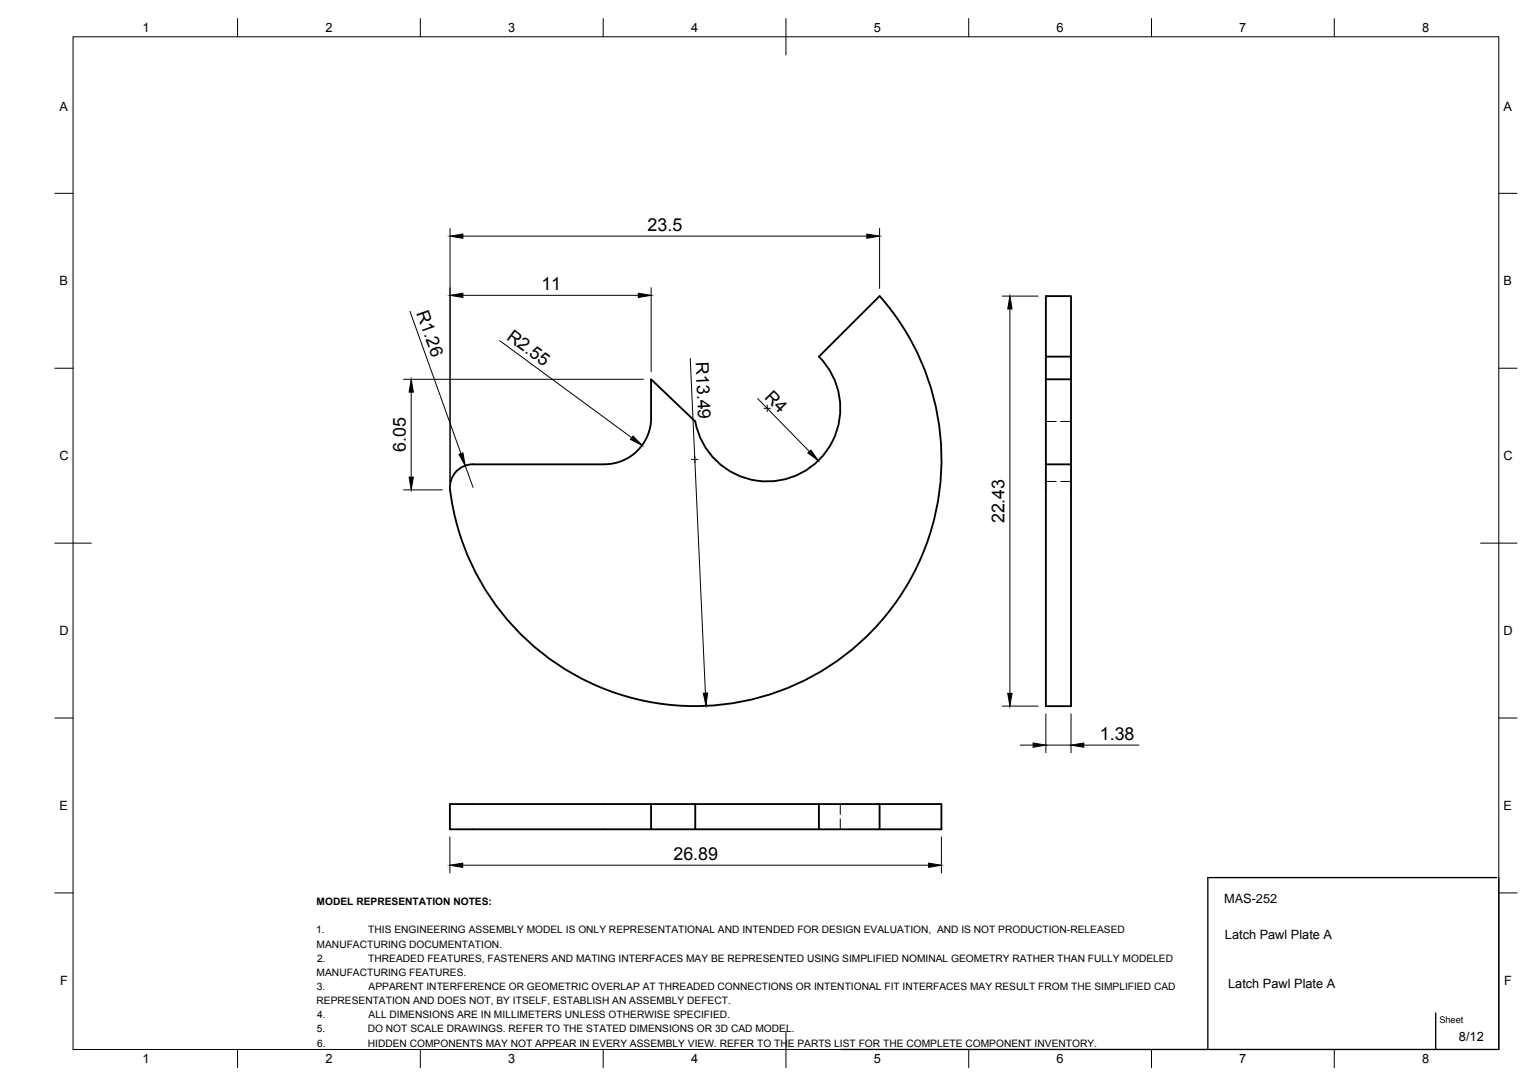
ISO-10303-21;
HEADER;
FILE_DESCRIPTION((''),'2;1');
FILE_NAME('Latch Pawl Plate A.step','2026-10-06T07:01:46+05:00',(''),(''),'','','');
FILE_SCHEMA (('AUTOMOTIVE_DESIGN { 1 0 10303 214 3 1 1 }'));
ENDSEC;
DATA;
#10=MECHANICAL_DESIGN_GEOMETRIC_PRESENTATION_REPRESENTATION('',(#150),#11396);
#120=SHAPE_REPRESENTATION_RELATIONSHIP('SRR','None',#11467,#135) ;
#135=ADVANCED_BREP_SHAPE_REPRESENTATION('',(#165),#11393) ;
#150=STYLED_ITEM('',(#11551),#165) ;
#165=MANIFOLD_SOLID_BREP('Latch Pawl Plate A',#5581) ;
#494=PLANE('',#6342) ;
#495=PLANE('',#6343) ;
#496=PLANE('',#6347) ;
#497=PLANE('',#6354) ;
#498=PLANE('',#6355) ;
#499=PLANE('',#6356) ;
#817=FACE_OUTER_BOUND('',#1190,.T.) ;
#818=FACE_OUTER_BOUND('',#1191,.T.) ;
#819=FACE_OUTER_BOUND('',#1192,.T.) ;
#820=FACE_OUTER_BOUND('',#1193,.T.) ;
#821=FACE_OUTER_BOUND('',#1194,.T.) ;
#822=FACE_OUTER_BOUND('',#1195,.T.) ;
#823=FACE_OUTER_BOUND('',#1196,.T.) ;
#824=FACE_OUTER_BOUND('',#1197,.T.) ;
#825=FACE_OUTER_BOUND('',#1198,.T.) ;
#826=FACE_OUTER_BOUND('',#1199,.T.) ;
#1190=EDGE_LOOP('',(#4966,#4967,#4968,#4969)) ;
#1191=EDGE_LOOP('',(#4970,#4971,#4972,#4973)) ;
#1192=EDGE_LOOP('',(#4974,#4975,#4976,#4977)) ;
#1193=EDGE_LOOP('',(#4978,#4979,#4980,#4981)) ;
#1194=EDGE_LOOP('',(#4982,#4983,#4984,#4985)) ;
#1195=EDGE_LOOP('',(#4986,#4987,#4988,#4989)) ;
#1196=EDGE_LOOP('',(#4990,#4991,#4992,#4993)) ;
#1197=EDGE_LOOP('',(#4994,#4995,#4996,#4997)) ;
#1198=EDGE_LOOP('',(#4998,#4999,#5000,#5001,#5002,#5003,#5004,#5005)) ;
#1199=EDGE_LOOP('',(#5006,#5007,#5008,#5009,#5010,#5011,#5012,#5013)) ;
#1567=LINE('',#11213,#1950) ;
#1568=LINE('',#11216,#1951) ;
#1569=LINE('',#11219,#1952) ;
#1570=LINE('',#11221,#1953) ;
#1571=LINE('',#11222,#1954) ;
#1572=LINE('',#11225,#1955) ;
#1573=LINE('',#11227,#1956) ;
#1574=LINE('',#11228,#1957) ;
#1575=LINE('',#11234,#1958) ;
#1576=LINE('',#11237,#1959) ;
#1577=LINE('',#11239,#1960) ;
#1578=LINE('',#11240,#1961) ;
#1579=LINE('',#11246,#1962) ;
#1580=LINE('',#11252,#1963) ;
#1581=LINE('',#11254,#1964) ;
#1582=LINE('',#11255,#1965) ;
#1950=VECTOR('',#7943,10.) ;
#1951=VECTOR('',#7946,10.) ;
#1952=VECTOR('',#7949,10.) ;
#1953=VECTOR('',#7950,10.) ;
#1954=VECTOR('',#7951,10.) ;
#1955=VECTOR('',#7954,10.) ;
#1956=VECTOR('',#7955,10.) ;
#1957=VECTOR('',#7956,10.) ;
#1958=VECTOR('',#7963,10.) ;
#1959=VECTOR('',#7966,10.) ;
#1960=VECTOR('',#7967,10.) ;
#1961=VECTOR('',#7968,10.) ;
#1962=VECTOR('',#7975,10.) ;
#1963=VECTOR('',#7982,10.) ;
#1964=VECTOR('',#7985,10.) ;
#1965=VECTOR('',#7986,10.) ;
#2243=CIRCLE('',#6340,2.55000000000001) ;
#2244=CIRCLE('',#6341,2.55000000000001) ;
#2245=CIRCLE('',#6345,4.00044834860818) ;
#2246=CIRCLE('',#6346,4.00044834860818) ;
#2247=CIRCLE('',#6349,13.4930018479188) ;
#2248=CIRCLE('',#6350,13.4930018479188) ;
#2249=CIRCLE('',#6352,1.26348906976575) ;
#2250=CIRCLE('',#6353,1.26348906976575) ;
#2704=VERTEX_POINT('',#11209) ;
#2705=VERTEX_POINT('',#11210) ;
#2706=VERTEX_POINT('',#11212) ;
#2707=VERTEX_POINT('',#11214) ;
#2708=VERTEX_POINT('',#11218) ;
#2709=VERTEX_POINT('',#11220) ;
#2710=VERTEX_POINT('',#11224) ;
#2711=VERTEX_POINT('',#11226) ;
#2712=VERTEX_POINT('',#11230) ;
#2713=VERTEX_POINT('',#11232) ;
#2714=VERTEX_POINT('',#11236) ;
#2715=VERTEX_POINT('',#11238) ;
#2716=VERTEX_POINT('',#11242) ;
#2717=VERTEX_POINT('',#11244) ;
#2718=VERTEX_POINT('',#11248) ;
#2719=VERTEX_POINT('',#11250) ;
#3465=EDGE_CURVE('',#2704,#2705,#2243,.T.) ;
#3466=EDGE_CURVE('',#2704,#2706,#1567,.T.) ;
#3467=EDGE_CURVE('',#2707,#2706,#2244,.T.) ;
#3468=EDGE_CURVE('',#2705,#2707,#1568,.T.) ;
#3469=EDGE_CURVE('',#2708,#2705,#1569,.T.) ;
#3470=EDGE_CURVE('',#2709,#2707,#1570,.T.) ;
#3471=EDGE_CURVE('',#2708,#2709,#1571,.T.) ;
#3472=EDGE_CURVE('',#2710,#2708,#1572,.T.) ;
#3473=EDGE_CURVE('',#2711,#2709,#1573,.T.) ;
#3474=EDGE_CURVE('',#2710,#2711,#1574,.T.) ;
#3475=EDGE_CURVE('',#2710,#2712,#2245,.T.) ;
#3476=EDGE_CURVE('',#2713,#2711,#2246,.T.) ;
#3477=EDGE_CURVE('',#2712,#2713,#1575,.T.) ;
#3478=EDGE_CURVE('',#2714,#2712,#1576,.T.) ;
#3479=EDGE_CURVE('',#2715,#2713,#1577,.T.) ;
#3480=EDGE_CURVE('',#2714,#2715,#1578,.T.) ;
#3481=EDGE_CURVE('',#2716,#2714,#2247,.T.) ;
#3482=EDGE_CURVE('',#2717,#2715,#2248,.T.) ;
#3483=EDGE_CURVE('',#2716,#2717,#1579,.T.) ;
#3484=EDGE_CURVE('',#2718,#2716,#2249,.T.) ;
#3485=EDGE_CURVE('',#2719,#2717,#2250,.T.) ;
#3486=EDGE_CURVE('',#2718,#2719,#1580,.T.) ;
#3487=EDGE_CURVE('',#2704,#2718,#1581,.T.) ;
#3488=EDGE_CURVE('',#2706,#2719,#1582,.T.) ;
#4966=ORIENTED_EDGE('',*,*,#3465,.F.) ;
#4967=ORIENTED_EDGE('',*,*,#3466,.T.) ;
#4968=ORIENTED_EDGE('',*,*,#3467,.F.) ;
#4969=ORIENTED_EDGE('',*,*,#3468,.F.) ;
#4970=ORIENTED_EDGE('',*,*,#3469,.T.) ;
#4971=ORIENTED_EDGE('',*,*,#3468,.T.) ;
#4972=ORIENTED_EDGE('',*,*,#3470,.F.) ;
#4973=ORIENTED_EDGE('',*,*,#3471,.F.) ;
#4974=ORIENTED_EDGE('',*,*,#3472,.T.) ;
#4975=ORIENTED_EDGE('',*,*,#3471,.T.) ;
#4976=ORIENTED_EDGE('',*,*,#3473,.F.) ;
#4977=ORIENTED_EDGE('',*,*,#3474,.F.) ;
#4978=ORIENTED_EDGE('',*,*,#3475,.F.) ;
#4979=ORIENTED_EDGE('',*,*,#3474,.T.) ;
#4980=ORIENTED_EDGE('',*,*,#3476,.F.) ;
#4981=ORIENTED_EDGE('',*,*,#3477,.F.) ;
#4982=ORIENTED_EDGE('',*,*,#3478,.T.) ;
#4983=ORIENTED_EDGE('',*,*,#3477,.T.) ;
#4984=ORIENTED_EDGE('',*,*,#3479,.F.) ;
#4985=ORIENTED_EDGE('',*,*,#3480,.F.) ;
#4986=ORIENTED_EDGE('',*,*,#3481,.T.) ;
#4987=ORIENTED_EDGE('',*,*,#3480,.T.) ;
#4988=ORIENTED_EDGE('',*,*,#3482,.F.) ;
#4989=ORIENTED_EDGE('',*,*,#3483,.F.) ;
#4990=ORIENTED_EDGE('',*,*,#3484,.T.) ;
#4991=ORIENTED_EDGE('',*,*,#3483,.T.) ;
#4992=ORIENTED_EDGE('',*,*,#3485,.F.) ;
#4993=ORIENTED_EDGE('',*,*,#3486,.F.) ;
#4994=ORIENTED_EDGE('',*,*,#3487,.T.) ;
#4995=ORIENTED_EDGE('',*,*,#3486,.T.) ;
#4996=ORIENTED_EDGE('',*,*,#3488,.F.) ;
#4997=ORIENTED_EDGE('',*,*,#3466,.F.) ;
#4998=ORIENTED_EDGE('',*,*,#3488,.T.) ;
#4999=ORIENTED_EDGE('',*,*,#3485,.T.) ;
#5000=ORIENTED_EDGE('',*,*,#3482,.T.) ;
#5001=ORIENTED_EDGE('',*,*,#3479,.T.) ;
#5002=ORIENTED_EDGE('',*,*,#3476,.T.) ;
#5003=ORIENTED_EDGE('',*,*,#3473,.T.) ;
#5004=ORIENTED_EDGE('',*,*,#3470,.T.) ;
#5005=ORIENTED_EDGE('',*,*,#3467,.T.) ;
#5006=ORIENTED_EDGE('',*,*,#3487,.F.) ;
#5007=ORIENTED_EDGE('',*,*,#3465,.T.) ;
#5008=ORIENTED_EDGE('',*,*,#3469,.F.) ;
#5009=ORIENTED_EDGE('',*,*,#3472,.F.) ;
#5010=ORIENTED_EDGE('',*,*,#3475,.T.) ;
#5011=ORIENTED_EDGE('',*,*,#3478,.F.) ;
#5012=ORIENTED_EDGE('',*,*,#3481,.F.) ;
#5013=ORIENTED_EDGE('',*,*,#3484,.F.) ;
#5220=CYLINDRICAL_SURFACE('',#6339,2.55000000000001) ;
#5221=CYLINDRICAL_SURFACE('',#6344,4.00044834860818) ;
#5222=CYLINDRICAL_SURFACE('',#6348,13.4930018479188) ;
#5223=CYLINDRICAL_SURFACE('',#6351,1.26348906976575) ;
#5542=ADVANCED_FACE('',(#817),#5220,.F.) ;
#5543=ADVANCED_FACE('',(#818),#494,.T.) ;
#5544=ADVANCED_FACE('',(#819),#495,.T.) ;
#5545=ADVANCED_FACE('',(#820),#5221,.F.) ;
#5546=ADVANCED_FACE('',(#821),#496,.T.) ;
#5547=ADVANCED_FACE('',(#822),#5222,.T.) ;
#5548=ADVANCED_FACE('',(#823),#5223,.T.) ;
#5549=ADVANCED_FACE('',(#824),#497,.T.) ;
#5550=ADVANCED_FACE('',(#825),#498,.T.) ;
#5551=ADVANCED_FACE('',(#826),#499,.F.) ;
#5581=CLOSED_SHELL('',(#5542,#5543,#5544,#5545,#5546,#5547,#5548,#5549,
#5550,#5551)) ;
#6338=AXIS2_PLACEMENT_3D('',#11207,#7937,#7938) ;
#6339=AXIS2_PLACEMENT_3D('',#11208,#7939,#7940) ;
#6340=AXIS2_PLACEMENT_3D('',#11211,#7941,#7942) ;
#6341=AXIS2_PLACEMENT_3D('',#11215,#7944,#7945) ;
#6342=AXIS2_PLACEMENT_3D('',#11217,#7947,#7948) ;
#6343=AXIS2_PLACEMENT_3D('',#11223,#7952,#7953) ;
#6344=AXIS2_PLACEMENT_3D('',#11229,#7957,#7958) ;
#6345=AXIS2_PLACEMENT_3D('',#11231,#7959,#7960) ;
#6346=AXIS2_PLACEMENT_3D('',#11233,#7961,#7962) ;
#6347=AXIS2_PLACEMENT_3D('',#11235,#7964,#7965) ;
#6348=AXIS2_PLACEMENT_3D('',#11241,#7969,#7970) ;
#6349=AXIS2_PLACEMENT_3D('',#11243,#7971,#7972) ;
#6350=AXIS2_PLACEMENT_3D('',#11245,#7973,#7974) ;
#6351=AXIS2_PLACEMENT_3D('',#11247,#7976,#7977) ;
#6352=AXIS2_PLACEMENT_3D('',#11249,#7978,#7979) ;
#6353=AXIS2_PLACEMENT_3D('',#11251,#7980,#7981) ;
#6354=AXIS2_PLACEMENT_3D('',#11253,#7983,#7984) ;
#6355=AXIS2_PLACEMENT_3D('',#11256,#7987,#7988) ;
#6356=AXIS2_PLACEMENT_3D('',#11257,#7989,#7990) ;
#7937=DIRECTION('axis',(0.,0.,1.)) ;
#7938=DIRECTION('refdir',(1.,0.,0.)) ;
#7939=DIRECTION('center_axis',(1.,0.,0.)) ;
#7940=DIRECTION('ref_axis',(0.,-1.,-6.96610525254997E-15)) ;
#7941=DIRECTION('center_axis',(1.,0.,0.)) ;
#7942=DIRECTION('ref_axis',(0.,-1.,-6.96610525254997E-15)) ;
#7943=DIRECTION('',(1.,0.,0.)) ;
#7944=DIRECTION('center_axis',(-1.,0.,0.)) ;
#7945=DIRECTION('ref_axis',(0.,-1.,-6.96610525254997E-15)) ;
#7946=DIRECTION('',(1.,0.,0.)) ;
#7947=DIRECTION('center_axis',(0.,0.,1.)) ;
#7948=DIRECTION('ref_axis',(0.,-1.,0.)) ;
#7949=DIRECTION('',(0.,-1.,0.)) ;
#7950=DIRECTION('',(0.,-1.,0.)) ;
#7951=DIRECTION('',(1.,0.,0.)) ;
#7952=DIRECTION('center_axis',(0.,0.72338954512527,-0.690440124850414)) ;
#7953=DIRECTION('ref_axis',(0.,0.690440124850414,0.72338954512527)) ;
#7954=DIRECTION('',(0.,0.690440124850414,0.72338954512527)) ;
#7955=DIRECTION('',(0.,0.690440124850414,0.72338954512527)) ;
#7956=DIRECTION('',(1.,0.,0.)) ;
#7957=DIRECTION('center_axis',(1.,0.,0.)) ;
#7958=DIRECTION('ref_axis',(0.,-0.885754641370607,-0.464153762551191)) ;
#7959=DIRECTION('center_axis',(1.,0.,0.)) ;
#7960=DIRECTION('ref_axis',(0.,-0.179181570317841,0.983816021854916)) ;
#7961=DIRECTION('center_axis',(-1.,0.,0.)) ;
#7962=DIRECTION('ref_axis',(0.,-0.179181570317841,0.983816021854916)) ;
#7963=DIRECTION('',(1.,0.,0.)) ;
#7964=DIRECTION('center_axis',(0.,0.708172501721611,0.70603945201763)) ;
#7965=DIRECTION('ref_axis',(0.,-0.70603945201763,0.708172501721611)) ;
#7966=DIRECTION('',(0.,-0.70603945201763,0.708172501721611)) ;
#7967=DIRECTION('',(0.,-0.70603945201763,0.708172501721611)) ;
#7968=DIRECTION('',(1.,0.,0.)) ;
#7969=DIRECTION('center_axis',(1.,0.,0.)) ;
#7970=DIRECTION('ref_axis',(0.,-0.911558251075126,-0.411170955804099)) ;
#7971=DIRECTION('center_axis',(1.,0.,0.)) ;
#7972=DIRECTION('ref_axis',(0.,-0.12333775780625,0.992364750230139)) ;
#7973=DIRECTION('center_axis',(1.,0.,0.)) ;
#7974=DIRECTION('ref_axis',(0.,-0.12333775780625,0.992364750230139)) ;
#7975=DIRECTION('',(1.,0.,0.)) ;
#7976=DIRECTION('center_axis',(1.,0.,0.)) ;
#7977=DIRECTION('ref_axis',(0.,0.999988378789617,0.00482102537998268)) ;
#7978=DIRECTION('center_axis',(1.,0.,0.)) ;
#7979=DIRECTION('ref_axis',(0.,0.999988378789617,0.00482102537998268)) ;
#7980=DIRECTION('center_axis',(1.,0.,0.)) ;
#7981=DIRECTION('ref_axis',(0.,0.999988378789617,0.00482102537998268)) ;
#7982=DIRECTION('',(1.,0.,0.)) ;
#7983=DIRECTION('center_axis',(0.,1.,0.)) ;
#7984=DIRECTION('ref_axis',(0.,0.,1.)) ;
#7985=DIRECTION('',(0.,0.,1.)) ;
#7986=DIRECTION('',(0.,0.,1.)) ;
#7987=DIRECTION('center_axis',(1.,0.,0.)) ;
#7988=DIRECTION('ref_axis',(0.,0.,-1.)) ;
#7989=DIRECTION('center_axis',(1.,0.,0.)) ;
#7990=DIRECTION('ref_axis',(0.,0.,-1.)) ;
#11207=CARTESIAN_POINT('',(0.,0.,0.)) ;
#11208=CARTESIAN_POINT('Origin',(-1.435,17.05,36.05)) ;
#11209=CARTESIAN_POINT('',(-1.435,14.5,36.05)) ;
#11210=CARTESIAN_POINT('',(-1.435,17.05,33.5)) ;
#11211=CARTESIAN_POINT('Origin',(-1.435,17.05,36.05)) ;
#11212=CARTESIAN_POINT('',(-0.0600000000000001,14.5,36.05)) ;
#11213=CARTESIAN_POINT('',(-1.435,14.5,36.05)) ;
#11214=CARTESIAN_POINT('',(-0.0600000000000001,17.05,33.5)) ;
#11215=CARTESIAN_POINT('Origin',(-0.0600000000000001,17.05,36.05)) ;
#11216=CARTESIAN_POINT('',(-1.435,17.05,33.5)) ;
#11217=CARTESIAN_POINT('Origin',(-1.435,19.15,33.5)) ;
#11218=CARTESIAN_POINT('',(-1.435,19.15,33.5)) ;
#11219=CARTESIAN_POINT('',(-1.435,19.15,33.5)) ;
#11220=CARTESIAN_POINT('',(-0.0600000000000001,19.15,33.5)) ;
#11221=CARTESIAN_POINT('',(-0.0600000000000001,19.15,33.5)) ;
#11222=CARTESIAN_POINT('',(-1.435,19.15,33.5)) ;
#11223=CARTESIAN_POINT('Origin',(-1.435,16.845,31.085)) ;
#11224=CARTESIAN_POINT('',(-1.435,16.845,31.085)) ;
#11225=CARTESIAN_POINT('',(-1.435,16.845,31.085)) ;
#11226=CARTESIAN_POINT('',(-0.0600000000000001,16.845,31.085)) ;
#11227=CARTESIAN_POINT('',(-0.0600000000000001,16.845,31.085)) ;
#11228=CARTESIAN_POINT('',(-1.435,16.845,31.085)) ;
#11229=CARTESIAN_POINT('Origin',(-1.435,17.561806617079,27.1492948200362)) ;
#11230=CARTESIAN_POINT('',(-1.435,20.39,24.32)) ;
#11231=CARTESIAN_POINT('Origin',(-1.435,17.561806617079,27.1492948200362)) ;
#11232=CARTESIAN_POINT('',(-0.0600000000000001,20.39,24.32)) ;
#11233=CARTESIAN_POINT('Origin',(-0.0600000000000001,17.561806617079,27.1492948200362)) ;
#11234=CARTESIAN_POINT('',(-1.435,20.39,24.32)) ;
#11235=CARTESIAN_POINT('Origin',(-1.435,23.7,21.)) ;
#11236=CARTESIAN_POINT('',(-1.435,23.7,21.)) ;
#11237=CARTESIAN_POINT('',(-1.435,23.7,21.)) ;
#11238=CARTESIAN_POINT('',(-0.0600000000000001,23.7,21.)) ;
#11239=CARTESIAN_POINT('',(-0.0600000000000001,23.7,21.)) ;
#11240=CARTESIAN_POINT('',(-1.435,23.7,21.)) ;
#11241=CARTESIAN_POINT('Origin',(-1.435,14.7641965939979,31.1100205913352)) ;
#11242=CARTESIAN_POINT('',(-1.435,13.1,44.5)) ;
#11243=CARTESIAN_POINT('Origin',(-1.435,14.7641965939979,31.1100205913352)) ;
#11244=CARTESIAN_POINT('',(-0.0600000000000001,13.1,44.5)) ;
#11245=CARTESIAN_POINT('Origin',(-0.0600000000000001,14.7641965939979,31.1100205913352)) ;
#11246=CARTESIAN_POINT('',(-1.435,13.1,44.5)) ;
#11247=CARTESIAN_POINT('Origin',(-1.435,13.2365256135065,43.2439086871273)) ;
#11248=CARTESIAN_POINT('',(-1.435,14.5,43.25)) ;
#11249=CARTESIAN_POINT('Origin',(-1.435,13.2365256135065,43.2439086871273)) ;
#11250=CARTESIAN_POINT('',(-0.0600000000000001,14.5,43.25)) ;
#11251=CARTESIAN_POINT('Origin',(-0.0600000000000001,13.2365256135065,43.2439086871273)) ;
#11252=CARTESIAN_POINT('',(-1.435,14.5,43.25)) ;
#11253=CARTESIAN_POINT('Origin',(-1.435,14.5,36.05)) ;
#11254=CARTESIAN_POINT('',(-1.435,14.5,36.05)) ;
#11255=CARTESIAN_POINT('',(-0.0600000000000001,14.5,36.05)) ;
#11256=CARTESIAN_POINT('Origin',(-0.0600000000000001,12.4855973730395,31.0622082501547)) ;
#11257=CARTESIAN_POINT('Origin',(-1.435,12.4855973730395,31.0622082501547)) ;
#11376=UNCERTAINTY_MEASURE_WITH_UNIT(LENGTH_MEASURE(0.01),#11397,
'DISTANCE_ACCURACY_VALUE',
'Maximum model space distance between geometric entities at asserted c
onnectivities') ;
#11379=UNCERTAINTY_MEASURE_WITH_UNIT(LENGTH_MEASURE(0.01),#11397,
'DISTANCE_ACCURACY_VALUE',
'Maximum model space distance between geometric entities at asserted c
onnectivities') ;
#11393=(
GEOMETRIC_REPRESENTATION_CONTEXT(3)
GLOBAL_UNCERTAINTY_ASSIGNED_CONTEXT((#11376))
GLOBAL_UNIT_ASSIGNED_CONTEXT((#11397,#11399,#11400))
REPRESENTATION_CONTEXT('','3D')
) ;
#11396=(
GEOMETRIC_REPRESENTATION_CONTEXT(3)
GLOBAL_UNCERTAINTY_ASSIGNED_CONTEXT((#11379))
GLOBAL_UNIT_ASSIGNED_CONTEXT((#11397,#11399,#11400))
REPRESENTATION_CONTEXT('','3D')
) ;
#11397=(
LENGTH_UNIT()
NAMED_UNIT(*)
SI_UNIT(.MILLI.,.METRE.)
) ;
#11399=(
NAMED_UNIT(*)
PLANE_ANGLE_UNIT()
SI_UNIT($,.RADIAN.)
) ;
#11400=(
NAMED_UNIT(*)
SI_UNIT($,.STERADIAN.)
SOLID_ANGLE_UNIT()
) ;
#11414=SHAPE_DEFINITION_REPRESENTATION(#11430,#11467) ;
#11430=PRODUCT_DEFINITION_SHAPE('',$,#11484) ;
#11467=SHAPE_REPRESENTATION('',(#6338),#11393) ;
#11470=PRODUCT_DEFINITION_CONTEXT('part definition',#11520,'design') ;
#11484=PRODUCT_DEFINITION('Latch Pawl Plate A',
'Latch Pawl Plate A',#11500,#11470) ;
#11500=PRODUCT_DEFINITION_FORMATION('',$,#11535) ;
#11520=APPLICATION_CONTEXT(
'Core Data for Automotive Mechanical Design Process') ;
#11521=PRODUCT_CONTEXT('part definition',#11520,'mechanical') ;
#11535=PRODUCT('Latch Pawl Plate A','Latch Pawl Plate A',$,(#11521)) ;
#11551=PRESENTATION_STYLE_ASSIGNMENT((#11567)) ;
#11567=SURFACE_STYLE_USAGE(.BOTH.,#11583) ;
#11583=SURFACE_SIDE_STYLE('',(#11599)) ;
#11599=SURFACE_STYLE_FILL_AREA(#11615) ;
#11615=FILL_AREA_STYLE('MAS-252 Metallic - Latch Pawl Plate A',(#11631)) ;
#11631=FILL_AREA_STYLE_COLOUR('MAS-252 Metallic - Latch Pawl Plate A',#11647) ;
#11647=COLOUR_RGB('MAS-252 Metallic - Latch Pawl Plate A', 0.09019608, 0.27058824, 0.51372549) ;
ENDSEC;
END-ISO-10303-21;
